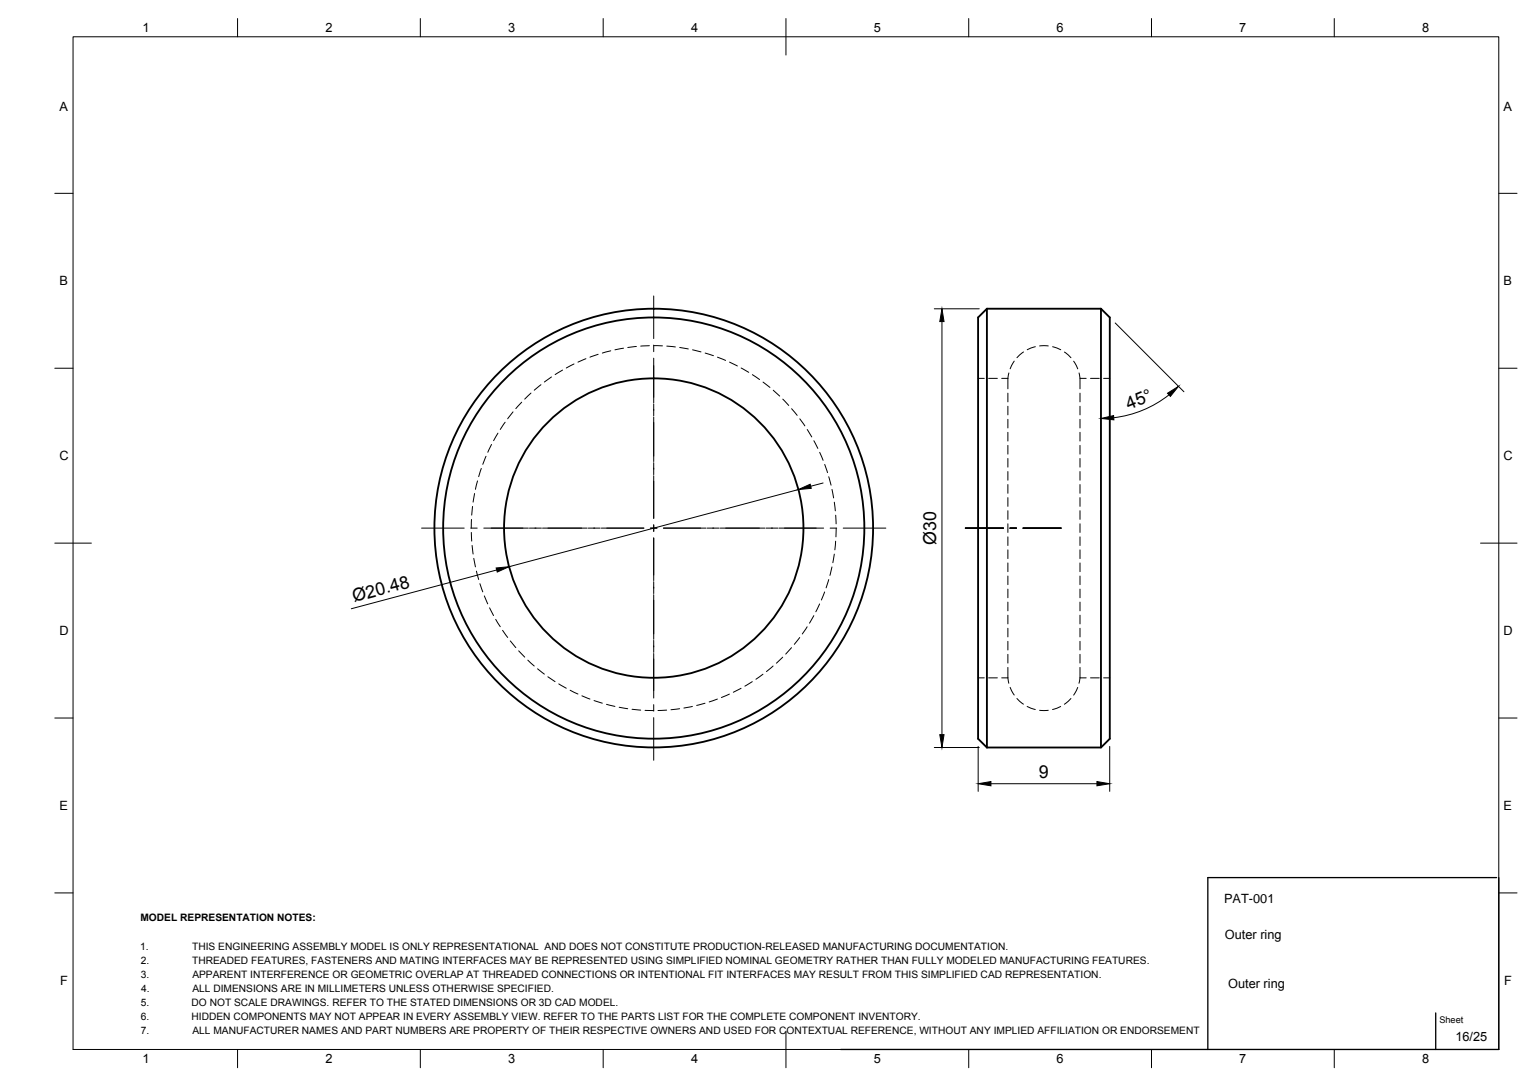
ISO-10303-21;
HEADER;
/* Generated by software containing ST-Developer
 * from STEP Tools, Inc. (www.steptools.com) 
 */

FILE_DESCRIPTION(
/* description */ ('PAT-001'),
/* implementation_level */ '2;1');

FILE_NAME(
/* name */ 'Outer ring.step',
/* time_stamp */ '2026-10-29T17:07:15-07:00',
/* author */ (''),
/* organization */ (''),
/* preprocessor_version */ 'ST-DEVELOPER v20.2',
/* originating_system */ 'Autodesk Translation Framework v15.17.0.0',
/* authorisation */ '');

FILE_SCHEMA (('AUTOMOTIVE_DESIGN { 1 0 10303 214 3 1 1 }'));
ENDSEC;

DATA;
#10=MECHANICAL_DESIGN_GEOMETRIC_PRESENTATION_REPRESENTATION('',(#379),#9622);
#307=CONICAL_SURFACE('',#5602,1.47,0.785398163397449);
#308=CONICAL_SURFACE('',#5606,1.47,0.785398163397449);
#322=TOROIDAL_SURFACE('',#5591,1.,0.247676);
#329=SHAPE_REPRESENTATION_RELATIONSHIP('SRR','None',#9753,#354);
#354=ADVANCED_BREP_SHAPE_REPRESENTATION('',(#412),#9602);
#379=STYLED_ITEM('',(#9962),#412);
#412=MANIFOLD_SOLID_BREP('Body1',#5204);
#451=FACE_BOUND('',#1063,.T.);
#452=FACE_BOUND('',#1068,.T.);
#544=PLANE('',#5599);
#545=PLANE('',#5608);
#750=FACE_OUTER_BOUND('',#1060,.T.);
#751=FACE_OUTER_BOUND('',#1061,.T.);
#752=FACE_OUTER_BOUND('',#1062,.T.);
#753=FACE_OUTER_BOUND('',#1064,.T.);
#754=FACE_OUTER_BOUND('',#1065,.T.);
#755=FACE_OUTER_BOUND('',#1066,.T.);
#756=FACE_OUTER_BOUND('',#1067,.T.);
#757=FACE_OUTER_BOUND('',#1069,.T.);
#1060=EDGE_LOOP('',(#3627,#3628,#3629,#3630,#3631,#3632));
#1061=EDGE_LOOP('',(#3633,#3634,#3635,#3636,#3637));
#1062=EDGE_LOOP('',(#3638));
#1063=EDGE_LOOP('',(#3639));
#1064=EDGE_LOOP('',(#3640,#3641,#3642,#3643));
#1065=EDGE_LOOP('',(#3644,#3645,#3646,#3647));
#1066=EDGE_LOOP('',(#3648,#3649,#3650,#3651));
#1067=EDGE_LOOP('',(#3652));
#1068=EDGE_LOOP('',(#3653));
#1069=EDGE_LOOP('',(#3654,#3655,#3656,#3657,#3658));
#1416=LINE('',#7857,#1821);
#1417=LINE('',#7866,#1822);
#1418=LINE('',#7870,#1823);
#1419=LINE('',#7874,#1824);
#1420=LINE('',#7877,#1825);
#1821=VECTOR('',#6305,1.023815);
#1822=VECTOR('',#6316,1.47);
#1823=VECTOR('',#6321,1.5);
#1824=VECTOR('',#6326,1.47);
#1825=VECTOR('',#6331,1.023815);
#2245=CIRCLE('',#5592,1.023815);
#2246=CIRCLE('',#5593,1.023815);
#2247=CIRCLE('',#5594,0.247676);
#2248=CIRCLE('',#5595,1.023815);
#2249=CIRCLE('',#5596,1.023815);
#2250=CIRCLE('',#5598,1.023815);
#2251=CIRCLE('',#5600,1.44);
#2252=CIRCLE('',#5601,1.023815);
#2253=CIRCLE('',#5603,1.5);
#2254=CIRCLE('',#5605,1.5);
#2255=CIRCLE('',#5607,1.44);
#2456=VERTEX_POINT('',#7845);
#2457=VERTEX_POINT('',#7846);
#2458=VERTEX_POINT('',#7849);
#2459=VERTEX_POINT('',#7851);
#2460=VERTEX_POINT('',#7855);
#2461=VERTEX_POINT('',#7859);
#2462=VERTEX_POINT('',#7861);
#2463=VERTEX_POINT('',#7864);
#2464=VERTEX_POINT('',#7868);
#2465=VERTEX_POINT('',#7872);
#2917=EDGE_CURVE('',#2456,#2457,#2245,.T.);
#2918=EDGE_CURVE('',#2457,#2456,#2246,.T.);
#2919=EDGE_CURVE('',#2457,#2458,#2247,.T.);
#2920=EDGE_CURVE('',#2459,#2458,#2248,.T.);
#2921=EDGE_CURVE('',#2458,#2459,#2249,.T.);
#2922=EDGE_CURVE('',#2460,#2460,#2250,.T.);
#2923=EDGE_CURVE('',#2460,#2459,#1416,.T.);
#2924=EDGE_CURVE('',#2461,#2461,#2251,.T.);
#2925=EDGE_CURVE('',#2462,#2462,#2252,.T.);
#2926=EDGE_CURVE('',#2463,#2463,#2253,.T.);
#2927=EDGE_CURVE('',#2463,#2461,#1417,.T.);
#2928=EDGE_CURVE('',#2464,#2464,#2254,.T.);
#2929=EDGE_CURVE('',#2464,#2463,#1418,.T.);
#2930=EDGE_CURVE('',#2465,#2465,#2255,.T.);
#2931=EDGE_CURVE('',#2465,#2464,#1419,.T.);
#2932=EDGE_CURVE('',#2456,#2462,#1420,.T.);
#3627=ORIENTED_EDGE('',*,*,#2917,.F.);
#3628=ORIENTED_EDGE('',*,*,#2918,.F.);
#3629=ORIENTED_EDGE('',*,*,#2919,.T.);
#3630=ORIENTED_EDGE('',*,*,#2920,.F.);
#3631=ORIENTED_EDGE('',*,*,#2921,.F.);
#3632=ORIENTED_EDGE('',*,*,#2919,.F.);
#3633=ORIENTED_EDGE('',*,*,#2922,.T.);
#3634=ORIENTED_EDGE('',*,*,#2923,.T.);
#3635=ORIENTED_EDGE('',*,*,#2920,.T.);
#3636=ORIENTED_EDGE('',*,*,#2921,.T.);
#3637=ORIENTED_EDGE('',*,*,#2923,.F.);
#3638=ORIENTED_EDGE('',*,*,#2924,.F.);
#3639=ORIENTED_EDGE('',*,*,#2925,.T.);
#3640=ORIENTED_EDGE('',*,*,#2926,.F.);
#3641=ORIENTED_EDGE('',*,*,#2927,.T.);
#3642=ORIENTED_EDGE('',*,*,#2924,.T.);
#3643=ORIENTED_EDGE('',*,*,#2927,.F.);
#3644=ORIENTED_EDGE('',*,*,#2928,.F.);
#3645=ORIENTED_EDGE('',*,*,#2929,.T.);
#3646=ORIENTED_EDGE('',*,*,#2926,.T.);
#3647=ORIENTED_EDGE('',*,*,#2929,.F.);
#3648=ORIENTED_EDGE('',*,*,#2930,.F.);
#3649=ORIENTED_EDGE('',*,*,#2931,.T.);
#3650=ORIENTED_EDGE('',*,*,#2928,.T.);
#3651=ORIENTED_EDGE('',*,*,#2931,.F.);
#3652=ORIENTED_EDGE('',*,*,#2930,.T.);
#3653=ORIENTED_EDGE('',*,*,#2922,.F.);
#3654=ORIENTED_EDGE('',*,*,#2917,.T.);
#3655=ORIENTED_EDGE('',*,*,#2918,.T.);
#3656=ORIENTED_EDGE('',*,*,#2932,.T.);
#3657=ORIENTED_EDGE('',*,*,#2925,.F.);
#3658=ORIENTED_EDGE('',*,*,#2932,.F.);
#4843=CYLINDRICAL_SURFACE('',#5597,1.023815);
#4844=CYLINDRICAL_SURFACE('',#5604,1.5);
#4845=CYLINDRICAL_SURFACE('',#5609,1.023815);
#4937=ADVANCED_FACE('',(#750),#322,.F.);
#4938=ADVANCED_FACE('',(#751),#4843,.F.);
#4939=ADVANCED_FACE('',(#752,#451),#544,.T.);
#4940=ADVANCED_FACE('',(#753),#307,.T.);
#4941=ADVANCED_FACE('',(#754),#4844,.T.);
#4942=ADVANCED_FACE('',(#755),#308,.T.);
#4943=ADVANCED_FACE('',(#756,#452),#545,.T.);
#4944=ADVANCED_FACE('',(#757),#4845,.F.);
#5204=CLOSED_SHELL('',(#4937,#4938,#4939,#4940,#4941,#4942,#4943,#4944));
#5590=AXIS2_PLACEMENT_3D('',#7843,#6287,#6288);
#5591=AXIS2_PLACEMENT_3D('',#7844,#6289,#6290);
#5592=AXIS2_PLACEMENT_3D('',#7847,#6291,#6292);
#5593=AXIS2_PLACEMENT_3D('',#7848,#6293,#6294);
#5594=AXIS2_PLACEMENT_3D('',#7850,#6295,#6296);
#5595=AXIS2_PLACEMENT_3D('',#7852,#6297,#6298);
#5596=AXIS2_PLACEMENT_3D('',#7853,#6299,#6300);
#5597=AXIS2_PLACEMENT_3D('',#7854,#6301,#6302);
#5598=AXIS2_PLACEMENT_3D('',#7856,#6303,#6304);
#5599=AXIS2_PLACEMENT_3D('',#7858,#6306,#6307);
#5600=AXIS2_PLACEMENT_3D('',#7860,#6308,#6309);
#5601=AXIS2_PLACEMENT_3D('',#7862,#6310,#6311);
#5602=AXIS2_PLACEMENT_3D('',#7863,#6312,#6313);
#5603=AXIS2_PLACEMENT_3D('',#7865,#6314,#6315);
#5604=AXIS2_PLACEMENT_3D('',#7867,#6317,#6318);
#5605=AXIS2_PLACEMENT_3D('',#7869,#6319,#6320);
#5606=AXIS2_PLACEMENT_3D('',#7871,#6322,#6323);
#5607=AXIS2_PLACEMENT_3D('',#7873,#6324,#6325);
#5608=AXIS2_PLACEMENT_3D('',#7875,#6327,#6328);
#5609=AXIS2_PLACEMENT_3D('',#7876,#6329,#6330);
#6287=DIRECTION('axis',(0.,0.,1.));
#6288=DIRECTION('refdir',(1.,0.,0.));
#6289=DIRECTION('center_axis',(0.,-1.,0.));
#6290=DIRECTION('ref_axis',(0.,0.,-1.));
#6291=DIRECTION('center_axis',(0.,-1.,0.));
#6292=DIRECTION('ref_axis',(1.,0.,0.));
#6293=DIRECTION('center_axis',(0.,-1.,0.));
#6294=DIRECTION('ref_axis',(1.,0.,0.));
#6295=DIRECTION('center_axis',(1.,0.,1.22464679914735E-16));
#6296=DIRECTION('ref_axis',(-1.22464679914735E-16,0.,1.));
#6297=DIRECTION('center_axis',(0.,1.,0.));
#6298=DIRECTION('ref_axis',(1.,0.,0.));
#6299=DIRECTION('center_axis',(0.,1.,0.));
#6300=DIRECTION('ref_axis',(1.,0.,0.));
#6301=DIRECTION('center_axis',(0.,-1.,0.));
#6302=DIRECTION('ref_axis',(1.,0.,0.));
#6303=DIRECTION('center_axis',(0.,-1.,0.));
#6304=DIRECTION('ref_axis',(1.,0.,0.));
#6305=DIRECTION('',(0.,1.,0.));
#6306=DIRECTION('center_axis',(0.,1.,0.));
#6307=DIRECTION('ref_axis',(0.,0.,1.));
#6308=DIRECTION('center_axis',(0.,-1.,0.));
#6309=DIRECTION('ref_axis',(1.,0.,0.));
#6310=DIRECTION('center_axis',(0.,-1.,0.));
#6311=DIRECTION('ref_axis',(1.,0.,0.));
#6312=DIRECTION('center_axis',(0.,-1.,0.));
#6313=DIRECTION('ref_axis',(1.,0.,0.));
#6314=DIRECTION('center_axis',(0.,-1.,0.));
#6315=DIRECTION('ref_axis',(1.,0.,0.));
#6316=DIRECTION('',(0.707106781186548,0.707106781186547,8.65956056235494E-17));
#6317=DIRECTION('center_axis',(0.,-1.,0.));
#6318=DIRECTION('ref_axis',(1.,0.,0.));
#6319=DIRECTION('center_axis',(0.,-1.,0.));
#6320=DIRECTION('ref_axis',(1.,0.,0.));
#6321=DIRECTION('',(0.,1.,0.));
#6322=DIRECTION('center_axis',(0.,1.,0.));
#6323=DIRECTION('ref_axis',(1.,0.,0.));
#6324=DIRECTION('center_axis',(0.,-1.,0.));
#6325=DIRECTION('ref_axis',(1.,0.,0.));
#6326=DIRECTION('',(-0.707106781186548,0.707106781186547,-8.65956056235494E-17));
#6327=DIRECTION('center_axis',(0.,-1.,0.));
#6328=DIRECTION('ref_axis',(0.,0.,-1.));
#6329=DIRECTION('center_axis',(0.,-1.,0.));
#6330=DIRECTION('ref_axis',(1.,0.,0.));
#6331=DIRECTION('',(0.,1.,0.));
#7843=CARTESIAN_POINT('',(0.,0.,0.));
#7844=CARTESIAN_POINT('Origin',(0.,0.,0.));
#7845=CARTESIAN_POINT('',(-1.023815,0.246528389340863,-1.25381176266905E-16));
#7846=CARTESIAN_POINT('',(-1.25381176266905E-16,0.246528389340863,1.023815));
#7847=CARTESIAN_POINT('Origin',(0.,0.246528389340863,0.));
#7848=CARTESIAN_POINT('Origin',(0.,0.246528389340863,0.));
#7849=CARTESIAN_POINT('',(-1.25381176266905E-16,-0.246528389340863,1.023815));
#7850=CARTESIAN_POINT('Origin',(-1.22464679914735E-16,0.,1.));
#7851=CARTESIAN_POINT('',(-1.023815,-0.246528389340863,1.25381176266905E-16));
#7852=CARTESIAN_POINT('Origin',(0.,-0.246528389340863,0.));
#7853=CARTESIAN_POINT('Origin',(0.,-0.246528389340863,0.));
#7854=CARTESIAN_POINT('Origin',(0.,0.,0.));
#7855=CARTESIAN_POINT('',(-1.023815,-0.45,-1.25381176266905E-16));
#7856=CARTESIAN_POINT('Origin',(0.,-0.45,0.));
#7857=CARTESIAN_POINT('',(-1.023815,0.,-1.25381176266905E-16));
#7858=CARTESIAN_POINT('Origin',(1.44,0.45,0.));
#7859=CARTESIAN_POINT('',(-1.44,0.45,-1.76349139077219E-16));
#7860=CARTESIAN_POINT('Origin',(0.,0.45,0.));
#7861=CARTESIAN_POINT('',(-1.023815,0.45,-1.25381176266905E-16));
#7862=CARTESIAN_POINT('Origin',(0.,0.45,0.));
#7863=CARTESIAN_POINT('Origin',(0.,0.42,0.));
#7864=CARTESIAN_POINT('',(-1.5,0.39,-1.83697019872103E-16));
#7865=CARTESIAN_POINT('Origin',(0.,0.39,0.));
#7866=CARTESIAN_POINT('',(-1.47,0.42,-1.80023079474661E-16));
#7867=CARTESIAN_POINT('Origin',(0.,0.,0.));
#7868=CARTESIAN_POINT('',(-1.5,-0.39,-1.83697019872103E-16));
#7869=CARTESIAN_POINT('Origin',(0.,-0.39,0.));
#7870=CARTESIAN_POINT('',(-1.5,0.,-1.83697019872103E-16));
#7871=CARTESIAN_POINT('Origin',(0.,-0.42,0.));
#7872=CARTESIAN_POINT('',(-1.44,-0.45,-1.76349139077219E-16));
#7873=CARTESIAN_POINT('Origin',(0.,-0.45,0.));
#7874=CARTESIAN_POINT('',(-1.47,-0.42,-1.80023079474661E-16));
#7875=CARTESIAN_POINT('Origin',(1.023815,-0.45,0.));
#7876=CARTESIAN_POINT('Origin',(0.,0.,0.));
#7877=CARTESIAN_POINT('',(-1.023815,0.,-1.25381176266905E-16));
#9572=UNCERTAINTY_MEASURE_WITH_UNIT(LENGTH_MEASURE(0.001),#9623,
'DISTANCE_ACCURACY_VALUE',
'Maximum model space distance between geometric entities at asserted c
onnectivities');
#9592=UNCERTAINTY_MEASURE_WITH_UNIT(LENGTH_MEASURE(0.001),#9623,
'DISTANCE_ACCURACY_VALUE',
'Maximum model space distance between geometric entities at asserted c
onnectivities');
#9602=(
GEOMETRIC_REPRESENTATION_CONTEXT(3)
GLOBAL_UNCERTAINTY_ASSIGNED_CONTEXT((#9572))
GLOBAL_UNIT_ASSIGNED_CONTEXT((#9623,#9625,#9626))
REPRESENTATION_CONTEXT('','3D')
);
#9622=(
GEOMETRIC_REPRESENTATION_CONTEXT(3)
GLOBAL_UNCERTAINTY_ASSIGNED_CONTEXT((#9592))
GLOBAL_UNIT_ASSIGNED_CONTEXT((#9623,#9625,#9626))
REPRESENTATION_CONTEXT('','3D')
);
#9623=(
LENGTH_UNIT()
NAMED_UNIT(*)
SI_UNIT(.CENTI.,.METRE.)
);
#9625=(
NAMED_UNIT(*)
PLANE_ANGLE_UNIT()
SI_UNIT($,.RADIAN.)
);
#9626=(
NAMED_UNIT(*)
SI_UNIT($,.STERADIAN.)
SOLID_ANGLE_UNIT()
);
#9636=SHAPE_DEFINITION_REPRESENTATION(#9665,#9753);
#9665=PRODUCT_DEFINITION_SHAPE('',$,#9783);
#9753=SHAPE_REPRESENTATION('',(#5590),#9602);
#9773=PRODUCT_DEFINITION_CONTEXT('part definition',#9862,'design');
#9783=PRODUCT_DEFINITION('Outer ring','Outer ring',#9812,#9773);
#9812=PRODUCT_DEFINITION_FORMATION('',$,#9873);
#9862=APPLICATION_CONTEXT(
'Core Data for Automotive Mechanical Design Process');
#9863=PRODUCT_CONTEXT('part definition',#9862,'mechanical');
#9873=PRODUCT('Outer ring','Outer ring','Outer ring',(#9863));
#9956=COLOUR_RGB('Grey',0.48,0.52,0.57);
#9957=FILL_AREA_STYLE_COLOUR('',#9956);
#9958=FILL_AREA_STYLE('',(#9957));
#9959=SURFACE_STYLE_FILL_AREA(#9958);
#9960=SURFACE_SIDE_STYLE('',(#9959));
#9961=SURFACE_STYLE_USAGE(.BOTH.,#9960);
#9962=PRESENTATION_STYLE_ASSIGNMENT((#9961));
ENDSEC;
END-ISO-10303-21;
